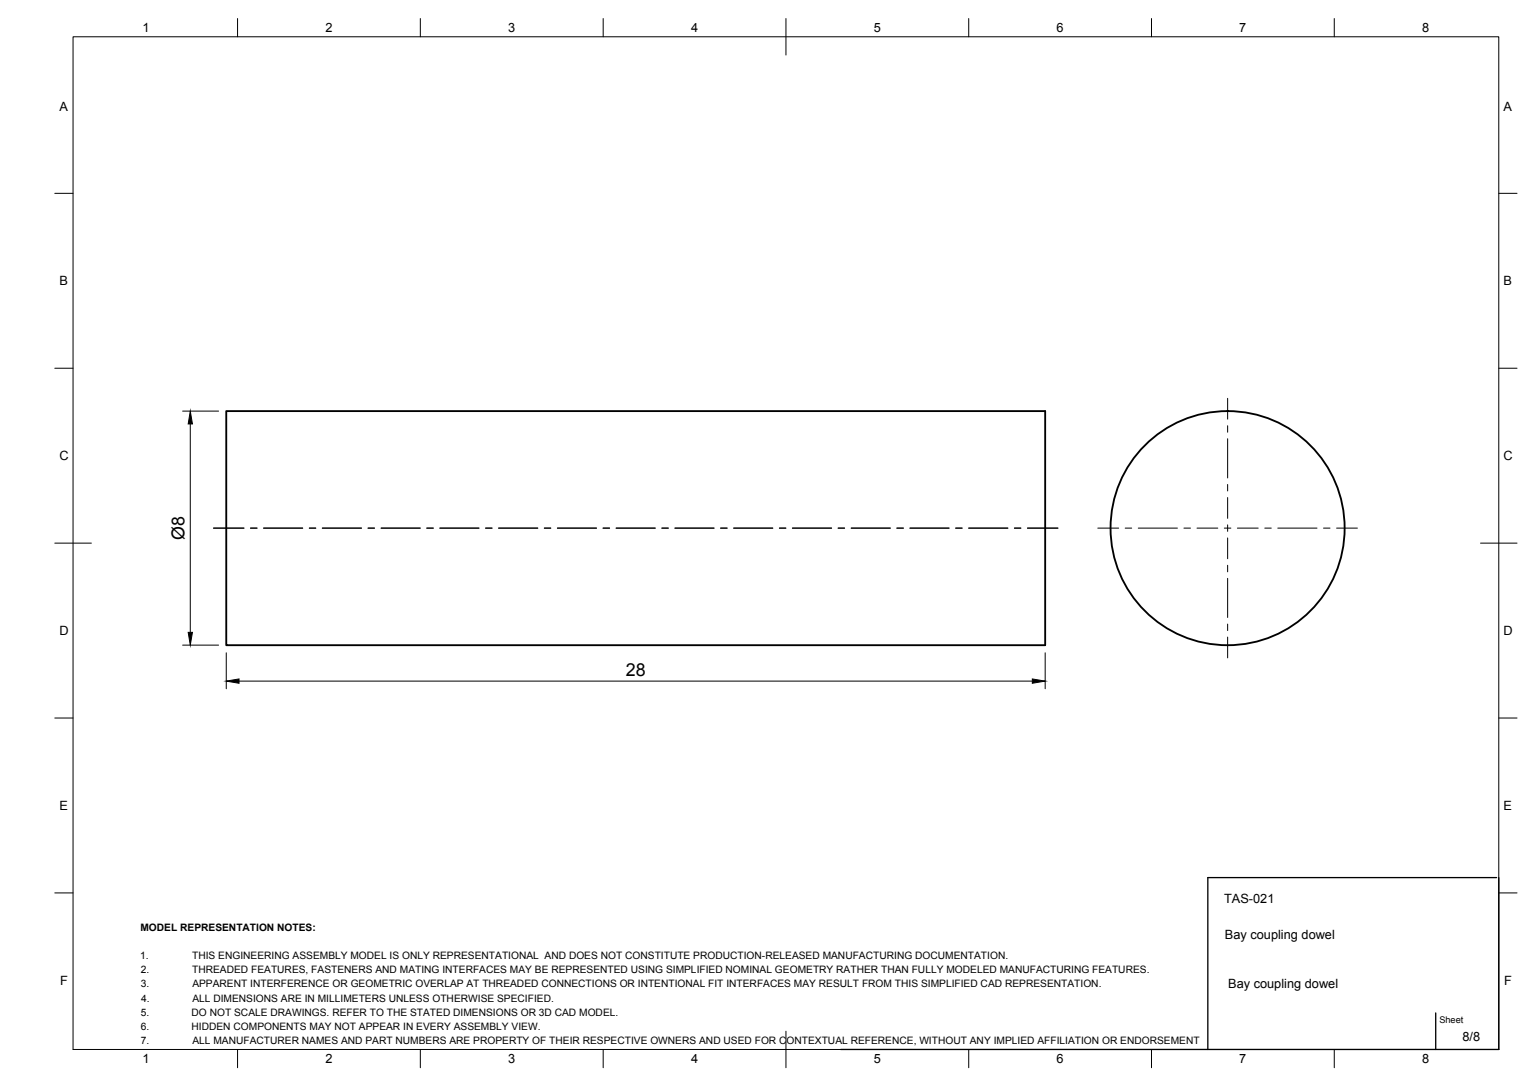
ISO-10303-21;
HEADER;
/* Generated by software containing ST-Developer
 * from STEP Tools, Inc. (www.steptools.com) 
 */

FILE_DESCRIPTION(
/* description */ (''),
/* implementation_level */ '2;1');

FILE_NAME(
/* name */ 'Bay coupling dowel.step',
/* time_stamp */ '2026-11-15T17:48:08-08:00',
/* author */ (''),
/* organization */ (''),
/* preprocessor_version */ 'ST-DEVELOPER v20.2',
/* originating_system */ 'Autodesk Translation Framework v15.17.0.0',
/* authorisation */ '');

FILE_SCHEMA (('AUTOMOTIVE_DESIGN { 1 0 10303 214 3 1 1 }'));
ENDSEC;

DATA;
#10=MECHANICAL_DESIGN_GEOMETRIC_PRESENTATION_REPRESENTATION('',(#144),#2097);
#132=SHAPE_REPRESENTATION_RELATIONSHIP('SRR','None',#2151,#138);
#138=ADVANCED_BREP_SHAPE_REPRESENTATION('',(#150),#2096);
#144=STYLED_ITEM('',(#2190),#150);
#150=MANIFOLD_SOLID_BREP('Body1',#1198);
#213=PLANE('',#1357);
#214=PLANE('',#1358);
#278=FACE_OUTER_BOUND('',#352,.T.);
#279=FACE_OUTER_BOUND('',#353,.T.);
#280=FACE_OUTER_BOUND('',#354,.T.);
#352=EDGE_LOOP('',(#1111,#1112,#1113,#1114));
#353=EDGE_LOOP('',(#1115));
#354=EDGE_LOOP('',(#1116));
#472=LINE('',#2049,#590);
#590=VECTOR('',#1685,0.4);
#609=CIRCLE('',#1355,0.4);
#610=CIRCLE('',#1356,0.4);
#701=VERTEX_POINT('',#2046);
#702=VERTEX_POINT('',#2048);
#838=EDGE_CURVE('',#701,#701,#609,.T.);
#839=EDGE_CURVE('',#701,#702,#472,.T.);
#840=EDGE_CURVE('',#702,#702,#610,.T.);
#1111=ORIENTED_EDGE('',*,*,#838,.F.);
#1112=ORIENTED_EDGE('',*,*,#839,.T.);
#1113=ORIENTED_EDGE('',*,*,#840,.T.);
#1114=ORIENTED_EDGE('',*,*,#839,.F.);
#1115=ORIENTED_EDGE('',*,*,#838,.T.);
#1116=ORIENTED_EDGE('',*,*,#840,.F.);
#1126=CYLINDRICAL_SURFACE('',#1354,0.4);
#1190=ADVANCED_FACE('',(#278),#1126,.T.);
#1191=ADVANCED_FACE('',(#279),#213,.T.);
#1192=ADVANCED_FACE('',(#280),#214,.F.);
#1198=CLOSED_SHELL('',(#1190,#1191,#1192));
#1353=AXIS2_PLACEMENT_3D('',#2044,#1679,#1680);
#1354=AXIS2_PLACEMENT_3D('',#2045,#1681,#1682);
#1355=AXIS2_PLACEMENT_3D('',#2047,#1683,#1684);
#1356=AXIS2_PLACEMENT_3D('',#2050,#1686,#1687);
#1357=AXIS2_PLACEMENT_3D('',#2051,#1688,#1689);
#1358=AXIS2_PLACEMENT_3D('',#2052,#1690,#1691);
#1679=DIRECTION('axis',(0.,0.,1.));
#1680=DIRECTION('refdir',(1.,0.,0.));
#1681=DIRECTION('center_axis',(0.,0.,1.));
#1682=DIRECTION('ref_axis',(1.,0.,0.));
#1683=DIRECTION('center_axis',(0.,0.,1.));
#1684=DIRECTION('ref_axis',(1.,0.,0.));
#1685=DIRECTION('',(0.,0.,-1.));
#1686=DIRECTION('center_axis',(0.,0.,1.));
#1687=DIRECTION('ref_axis',(1.,0.,0.));
#1688=DIRECTION('center_axis',(0.,0.,1.));
#1689=DIRECTION('ref_axis',(1.,0.,0.));
#1690=DIRECTION('center_axis',(0.,0.,1.));
#1691=DIRECTION('ref_axis',(1.,0.,0.));
#2044=CARTESIAN_POINT('',(0.,0.,0.));
#2045=CARTESIAN_POINT('Origin',(0.,0.,0.));
#2046=CARTESIAN_POINT('',(-0.4,-4.89858719658941E-17,2.8));
#2047=CARTESIAN_POINT('Origin',(0.,0.,2.8));
#2048=CARTESIAN_POINT('',(-0.4,-4.89858719658941E-17,0.));
#2049=CARTESIAN_POINT('',(-0.4,-4.89858719658941E-17,0.));
#2050=CARTESIAN_POINT('Origin',(0.,0.,0.));
#2051=CARTESIAN_POINT('Origin',(0.,0.,2.8));
#2052=CARTESIAN_POINT('Origin',(0.,0.,0.));
#2088=UNCERTAINTY_MEASURE_WITH_UNIT(LENGTH_MEASURE(0.001),#2098,
'DISTANCE_ACCURACY_VALUE',
'Maximum model space distance between geometric entities at asserted c
onnectivities');
#2089=UNCERTAINTY_MEASURE_WITH_UNIT(LENGTH_MEASURE(0.001),#2098,
'DISTANCE_ACCURACY_VALUE',
'Maximum model space distance between geometric entities at asserted c
onnectivities');
#2096=(
GEOMETRIC_REPRESENTATION_CONTEXT(3)
GLOBAL_UNCERTAINTY_ASSIGNED_CONTEXT((#2088))
GLOBAL_UNIT_ASSIGNED_CONTEXT((#2098,#2100,#2101))
REPRESENTATION_CONTEXT('','3D')
);
#2097=(
GEOMETRIC_REPRESENTATION_CONTEXT(3)
GLOBAL_UNCERTAINTY_ASSIGNED_CONTEXT((#2089))
GLOBAL_UNIT_ASSIGNED_CONTEXT((#2098,#2100,#2101))
REPRESENTATION_CONTEXT('','3D')
);
#2098=(
LENGTH_UNIT()
NAMED_UNIT(*)
SI_UNIT(.CENTI.,.METRE.)
);
#2100=(
NAMED_UNIT(*)
PLANE_ANGLE_UNIT()
SI_UNIT($,.RADIAN.)
);
#2101=(
NAMED_UNIT(*)
SI_UNIT($,.STERADIAN.)
SOLID_ANGLE_UNIT()
);
#2108=SHAPE_DEFINITION_REPRESENTATION(#2115,#2151);
#2115=PRODUCT_DEFINITION_SHAPE('',$,#2159);
#2151=SHAPE_REPRESENTATION('',(#1353),#2096);
#2152=PRODUCT_DEFINITION_CONTEXT('part definition',#2175,'design');
#2159=PRODUCT_DEFINITION('Bay coupling dowel','Bay coupling dowel',#2166,
#2152);
#2166=PRODUCT_DEFINITION_FORMATION('',$,#2183);
#2175=APPLICATION_CONTEXT(
'Core Data for Automotive Mechanical Design Process');
#2176=PRODUCT_CONTEXT('part definition',#2175,'mechanical');
#2183=PRODUCT('Bay coupling dowel','Bay coupling dowel',$,(#2176));
#2190=PRESENTATION_STYLE_ASSIGNMENT((#2197));
#2197=SURFACE_STYLE_USAGE(.BOTH.,#2204);
#2204=SURFACE_SIDE_STYLE('',(#2211));
#2211=SURFACE_STYLE_FILL_AREA(#2218);
#2218=FILL_AREA_STYLE('Bay coupling dowel finish',(#2225));
#2225=FILL_AREA_STYLE_COLOUR('Bay coupling dowel finish',#2232);
#2232=COLOUR_RGB('Bay coupling dowel finish',0.43921568627451,0.47843137254902,
0.52156862745098);
ENDSEC;
END-ISO-10303-21;
